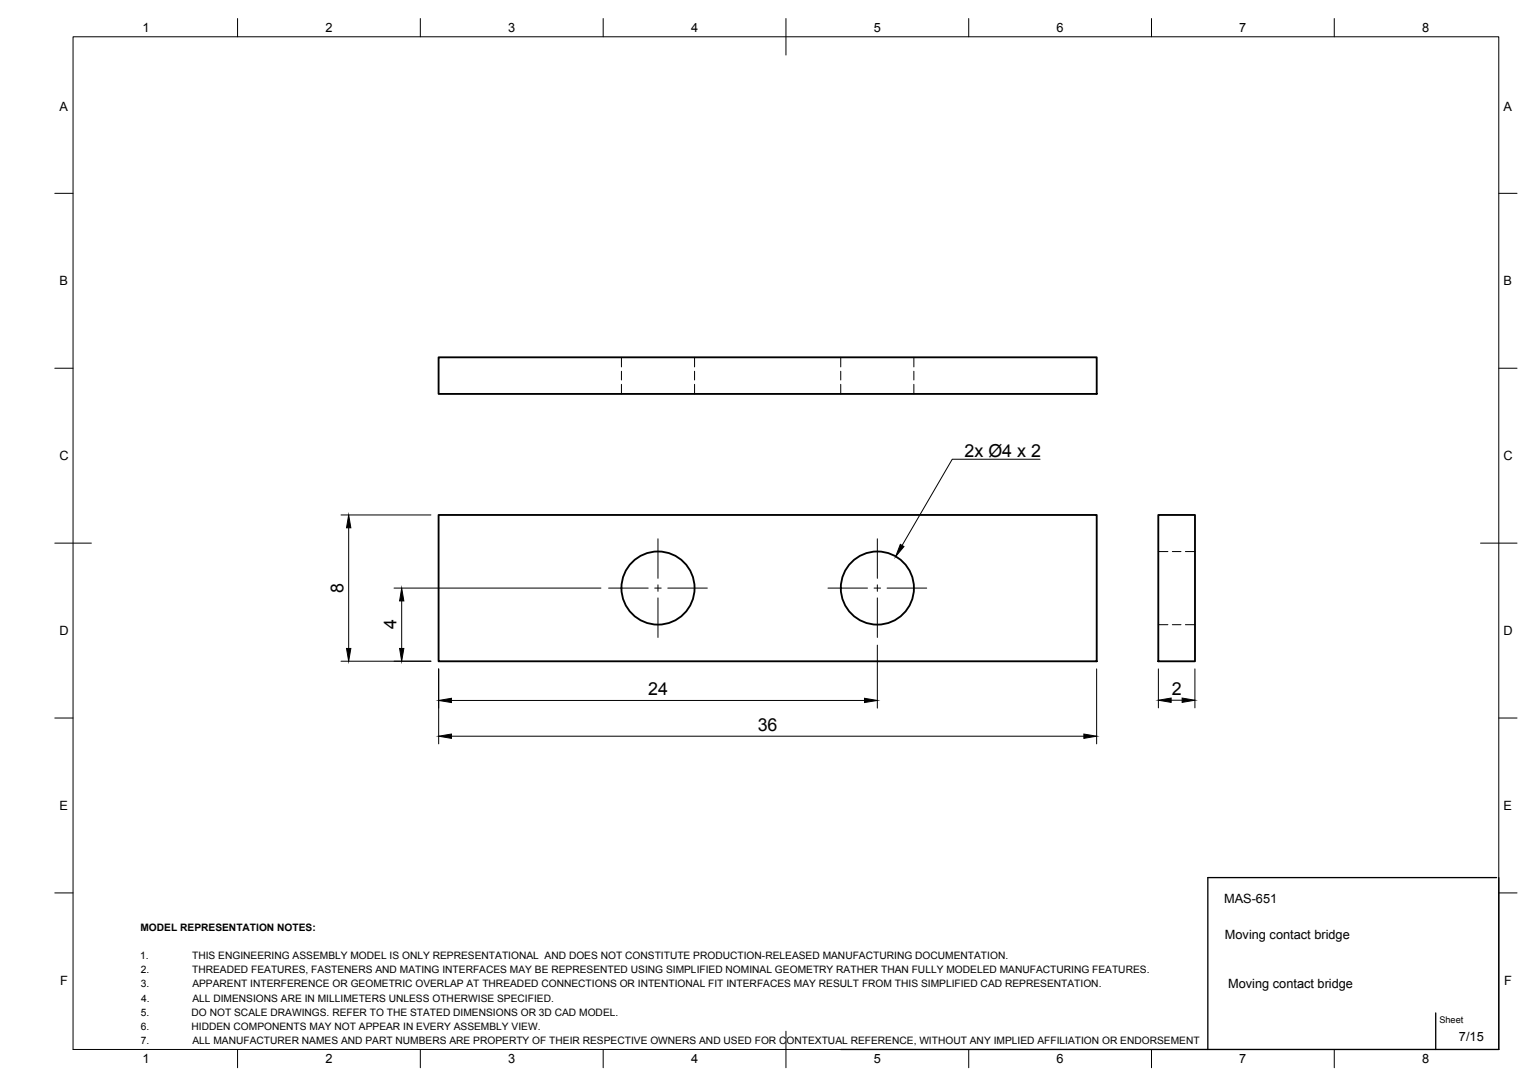
ISO-10303-21;
HEADER;
/* Generated by software containing ST-Developer
 * from STEP Tools, Inc. (www.steptools.com) 
 */

FILE_DESCRIPTION(
/* description */ ('Independent direct-acting normally-closed roller-plunger limit-switch
 CAD. Removable cover, insulated terminal supports, captured bus/conta
ct bridge, native Coil return spring, integral lower travel stop, reus
able instanced hardware and free roller. Manual geometric contact open
ing4mm; no snap-action/contact-force, electrical/current/voltage, envi
ronmental seal, safety-switch, wear, load or life certification. Exter
nal wiring and anchors omitted; fits and application engineering requi
red.'),
/* implementation_level */ '2;1');

FILE_NAME(
/* name */ 'Moving contact bridge.step',
/* time_stamp */ '2026-11-08T07:32:43-08:00',
/* author */ (''),
/* organization */ (''),
/* preprocessor_version */ 'ST-DEVELOPER v20.2',
/* originating_system */ 'Autodesk Translation Framework v15.17.0.0',
/* authorisation */ '');

FILE_SCHEMA (('AUTOMOTIVE_DESIGN { 1 0 10303 214 3 1 1 }'));
ENDSEC;

DATA;
#10=MECHANICAL_DESIGN_GEOMETRIC_PRESENTATION_REPRESENTATION('',(#180),#36482);
#146=SHAPE_REPRESENTATION_RELATIONSHIP('SRR','None',#36559,#163);
#163=ADVANCED_BREP_SHAPE_REPRESENTATION('',(#197),#36469);
#180=STYLED_ITEM('',(#36653),#197);
#197=MANIFOLD_SOLID_BREP('Body1',#9771);
#276=FACE_BOUND('',#1264,.T.);
#277=FACE_BOUND('',#1265,.T.);
#278=FACE_BOUND('',#1267,.T.);
#279=FACE_BOUND('',#1268,.T.);
#360=PLANE('',#10291);
#361=PLANE('',#10292);
#362=PLANE('',#10293);
#363=PLANE('',#10294);
#364=PLANE('',#10295);
#365=PLANE('',#10296);
#678=FACE_OUTER_BOUND('',#1257,.T.);
#679=FACE_OUTER_BOUND('',#1258,.T.);
#680=FACE_OUTER_BOUND('',#1259,.T.);
#681=FACE_OUTER_BOUND('',#1260,.T.);
#682=FACE_OUTER_BOUND('',#1261,.T.);
#683=FACE_OUTER_BOUND('',#1262,.T.);
#684=FACE_OUTER_BOUND('',#1263,.T.);
#685=FACE_OUTER_BOUND('',#1266,.T.);
#1257=EDGE_LOOP('',(#7302,#7303,#7304,#7305));
#1258=EDGE_LOOP('',(#7306,#7307,#7308,#7309));
#1259=EDGE_LOOP('',(#7310,#7311,#7312,#7313));
#1260=EDGE_LOOP('',(#7314,#7315,#7316,#7317));
#1261=EDGE_LOOP('',(#7318,#7319,#7320,#7321));
#1262=EDGE_LOOP('',(#7322,#7323,#7324,#7325));
#1263=EDGE_LOOP('',(#7326,#7327,#7328,#7329));
#1264=EDGE_LOOP('',(#7330));
#1265=EDGE_LOOP('',(#7331));
#1266=EDGE_LOOP('',(#7332,#7333,#7334,#7335));
#1267=EDGE_LOOP('',(#7336));
#1268=EDGE_LOOP('',(#7337));
#1662=CIRCLE('',#10286,0.2);
#1663=CIRCLE('',#10287,0.2);
#1664=CIRCLE('',#10289,0.2);
#1665=CIRCLE('',#10290,0.2);
#2707=LINE('',#23141,#3281);
#2708=LINE('',#23147,#3282);
#2709=LINE('',#23152,#3283);
#2710=LINE('',#23154,#3284);
#2711=LINE('',#23156,#3285);
#2712=LINE('',#23157,#3286);
#2713=LINE('',#23160,#3287);
#2714=LINE('',#23162,#3288);
#2715=LINE('',#23163,#3289);
#2716=LINE('',#23166,#3290);
#2717=LINE('',#23168,#3291);
#2718=LINE('',#23169,#3292);
#2719=LINE('',#23171,#3293);
#2720=LINE('',#23172,#3294);
#3281=VECTOR('',#11582,0.2);
#3282=VECTOR('',#11589,0.2);
#3283=VECTOR('',#11594,1.);
#3284=VECTOR('',#11595,1.);
#3285=VECTOR('',#11596,1.);
#3286=VECTOR('',#11597,1.);
#3287=VECTOR('',#11600,1.);
#3288=VECTOR('',#11601,1.);
#3289=VECTOR('',#11602,1.);
#3290=VECTOR('',#11605,1.);
#3291=VECTOR('',#11606,1.);
#3292=VECTOR('',#11607,1.);
#3293=VECTOR('',#11610,1.);
#3294=VECTOR('',#11611,1.);
#4031=VERTEX_POINT('',#23138);
#4032=VERTEX_POINT('',#23140);
#4033=VERTEX_POINT('',#23144);
#4034=VERTEX_POINT('',#23146);
#4035=VERTEX_POINT('',#23150);
#4036=VERTEX_POINT('',#23151);
#4037=VERTEX_POINT('',#23153);
#4038=VERTEX_POINT('',#23155);
#4039=VERTEX_POINT('',#23159);
#4040=VERTEX_POINT('',#23161);
#4041=VERTEX_POINT('',#23165);
#4042=VERTEX_POINT('',#23167);
#5207=EDGE_CURVE('',#4031,#4031,#1662,.T.);
#5208=EDGE_CURVE('',#4031,#4032,#2707,.T.);
#5209=EDGE_CURVE('',#4032,#4032,#1663,.T.);
#5210=EDGE_CURVE('',#4033,#4033,#1664,.T.);
#5211=EDGE_CURVE('',#4033,#4034,#2708,.T.);
#5212=EDGE_CURVE('',#4034,#4034,#1665,.T.);
#5213=EDGE_CURVE('',#4035,#4036,#2709,.T.);
#5214=EDGE_CURVE('',#4036,#4037,#2710,.T.);
#5215=EDGE_CURVE('',#4038,#4037,#2711,.T.);
#5216=EDGE_CURVE('',#4035,#4038,#2712,.T.);
#5217=EDGE_CURVE('',#4039,#4035,#2713,.T.);
#5218=EDGE_CURVE('',#4040,#4038,#2714,.T.);
#5219=EDGE_CURVE('',#4039,#4040,#2715,.T.);
#5220=EDGE_CURVE('',#4041,#4039,#2716,.T.);
#5221=EDGE_CURVE('',#4042,#4040,#2717,.T.);
#5222=EDGE_CURVE('',#4041,#4042,#2718,.T.);
#5223=EDGE_CURVE('',#4036,#4041,#2719,.T.);
#5224=EDGE_CURVE('',#4037,#4042,#2720,.T.);
#7302=ORIENTED_EDGE('',*,*,#5207,.F.);
#7303=ORIENTED_EDGE('',*,*,#5208,.T.);
#7304=ORIENTED_EDGE('',*,*,#5209,.F.);
#7305=ORIENTED_EDGE('',*,*,#5208,.F.);
#7306=ORIENTED_EDGE('',*,*,#5210,.F.);
#7307=ORIENTED_EDGE('',*,*,#5211,.T.);
#7308=ORIENTED_EDGE('',*,*,#5212,.F.);
#7309=ORIENTED_EDGE('',*,*,#5211,.F.);
#7310=ORIENTED_EDGE('',*,*,#5213,.T.);
#7311=ORIENTED_EDGE('',*,*,#5214,.T.);
#7312=ORIENTED_EDGE('',*,*,#5215,.F.);
#7313=ORIENTED_EDGE('',*,*,#5216,.F.);
#7314=ORIENTED_EDGE('',*,*,#5217,.T.);
#7315=ORIENTED_EDGE('',*,*,#5216,.T.);
#7316=ORIENTED_EDGE('',*,*,#5218,.F.);
#7317=ORIENTED_EDGE('',*,*,#5219,.F.);
#7318=ORIENTED_EDGE('',*,*,#5220,.T.);
#7319=ORIENTED_EDGE('',*,*,#5219,.T.);
#7320=ORIENTED_EDGE('',*,*,#5221,.F.);
#7321=ORIENTED_EDGE('',*,*,#5222,.F.);
#7322=ORIENTED_EDGE('',*,*,#5223,.T.);
#7323=ORIENTED_EDGE('',*,*,#5222,.T.);
#7324=ORIENTED_EDGE('',*,*,#5224,.F.);
#7325=ORIENTED_EDGE('',*,*,#5214,.F.);
#7326=ORIENTED_EDGE('',*,*,#5224,.T.);
#7327=ORIENTED_EDGE('',*,*,#5221,.T.);
#7328=ORIENTED_EDGE('',*,*,#5218,.T.);
#7329=ORIENTED_EDGE('',*,*,#5215,.T.);
#7330=ORIENTED_EDGE('',*,*,#5207,.T.);
#7331=ORIENTED_EDGE('',*,*,#5210,.T.);
#7332=ORIENTED_EDGE('',*,*,#5223,.F.);
#7333=ORIENTED_EDGE('',*,*,#5213,.F.);
#7334=ORIENTED_EDGE('',*,*,#5217,.F.);
#7335=ORIENTED_EDGE('',*,*,#5220,.F.);
#7336=ORIENTED_EDGE('',*,*,#5209,.T.);
#7337=ORIENTED_EDGE('',*,*,#5212,.T.);
#9029=CYLINDRICAL_SURFACE('',#10285,0.2);
#9030=CYLINDRICAL_SURFACE('',#10288,0.2);
#9468=ADVANCED_FACE('',(#678),#9029,.F.);
#9469=ADVANCED_FACE('',(#679),#9030,.F.);
#9470=ADVANCED_FACE('',(#680),#360,.T.);
#9471=ADVANCED_FACE('',(#681),#361,.T.);
#9472=ADVANCED_FACE('',(#682),#362,.T.);
#9473=ADVANCED_FACE('',(#683),#363,.T.);
#9474=ADVANCED_FACE('',(#684,#276,#277),#364,.T.);
#9475=ADVANCED_FACE('',(#685,#278,#279),#365,.F.);
#9771=CLOSED_SHELL('',(#9468,#9469,#9470,#9471,#9472,#9473,#9474,#9475));
#10284=AXIS2_PLACEMENT_3D('',#23136,#11576,#11577);
#10285=AXIS2_PLACEMENT_3D('',#23137,#11578,#11579);
#10286=AXIS2_PLACEMENT_3D('',#23139,#11580,#11581);
#10287=AXIS2_PLACEMENT_3D('',#23142,#11583,#11584);
#10288=AXIS2_PLACEMENT_3D('',#23143,#11585,#11586);
#10289=AXIS2_PLACEMENT_3D('',#23145,#11587,#11588);
#10290=AXIS2_PLACEMENT_3D('',#23148,#11590,#11591);
#10291=AXIS2_PLACEMENT_3D('',#23149,#11592,#11593);
#10292=AXIS2_PLACEMENT_3D('',#23158,#11598,#11599);
#10293=AXIS2_PLACEMENT_3D('',#23164,#11603,#11604);
#10294=AXIS2_PLACEMENT_3D('',#23170,#11608,#11609);
#10295=AXIS2_PLACEMENT_3D('',#23173,#11612,#11613);
#10296=AXIS2_PLACEMENT_3D('',#23174,#11614,#11615);
#11576=DIRECTION('axis',(0.,0.,1.));
#11577=DIRECTION('refdir',(1.,0.,0.));
#11578=DIRECTION('center_axis',(0.,0.,-1.));
#11579=DIRECTION('ref_axis',(1.,0.,0.));
#11580=DIRECTION('center_axis',(0.,0.,-1.));
#11581=DIRECTION('ref_axis',(1.,0.,0.));
#11582=DIRECTION('',(0.,0.,-1.));
#11583=DIRECTION('center_axis',(0.,0.,1.));
#11584=DIRECTION('ref_axis',(1.,0.,0.));
#11585=DIRECTION('center_axis',(0.,0.,-1.));
#11586=DIRECTION('ref_axis',(1.,0.,0.));
#11587=DIRECTION('center_axis',(0.,0.,-1.));
#11588=DIRECTION('ref_axis',(1.,0.,0.));
#11589=DIRECTION('',(0.,0.,-1.));
#11590=DIRECTION('center_axis',(0.,0.,1.));
#11591=DIRECTION('ref_axis',(1.,0.,0.));
#11592=DIRECTION('center_axis',(0.,1.,0.));
#11593=DIRECTION('ref_axis',(-1.,0.,0.));
#11594=DIRECTION('',(-1.,0.,0.));
#11595=DIRECTION('',(0.,0.,1.));
#11596=DIRECTION('',(-1.,0.,0.));
#11597=DIRECTION('',(0.,0.,1.));
#11598=DIRECTION('center_axis',(1.,0.,0.));
#11599=DIRECTION('ref_axis',(0.,1.,0.));
#11600=DIRECTION('',(0.,1.,0.));
#11601=DIRECTION('',(0.,1.,0.));
#11602=DIRECTION('',(0.,0.,1.));
#11603=DIRECTION('center_axis',(0.,-1.,0.));
#11604=DIRECTION('ref_axis',(1.,0.,0.));
#11605=DIRECTION('',(1.,0.,0.));
#11606=DIRECTION('',(1.,0.,0.));
#11607=DIRECTION('',(0.,0.,1.));
#11608=DIRECTION('center_axis',(-1.,0.,0.));
#11609=DIRECTION('ref_axis',(0.,-1.,0.));
#11610=DIRECTION('',(0.,-1.,0.));
#11611=DIRECTION('',(0.,-1.,0.));
#11612=DIRECTION('center_axis',(0.,0.,1.));
#11613=DIRECTION('ref_axis',(1.,0.,0.));
#11614=DIRECTION('center_axis',(0.,0.,1.));
#11615=DIRECTION('ref_axis',(1.,0.,0.));
#23136=CARTESIAN_POINT('',(0.,0.,0.));
#23137=CARTESIAN_POINT('Origin',(-0.6,1.,2.5));
#23138=CARTESIAN_POINT('',(-0.8,1.,2.6));
#23139=CARTESIAN_POINT('Origin',(-0.6,1.,2.6));
#23140=CARTESIAN_POINT('',(-0.8,1.,2.4));
#23141=CARTESIAN_POINT('',(-0.8,1.,2.5));
#23142=CARTESIAN_POINT('Origin',(-0.6,1.,2.4));
#23143=CARTESIAN_POINT('Origin',(0.6,1.,2.5));
#23144=CARTESIAN_POINT('',(0.4,1.,2.6));
#23145=CARTESIAN_POINT('Origin',(0.6,1.,2.6));
#23146=CARTESIAN_POINT('',(0.4,1.,2.4));
#23147=CARTESIAN_POINT('',(0.4,1.,2.5));
#23148=CARTESIAN_POINT('Origin',(0.6,1.,2.4));
#23149=CARTESIAN_POINT('Origin',(1.8,1.4,2.4));
#23150=CARTESIAN_POINT('',(1.8,1.4,2.4));
#23151=CARTESIAN_POINT('',(-1.8,1.4,2.4));
#23152=CARTESIAN_POINT('',(1.8,1.4,2.4));
#23153=CARTESIAN_POINT('',(-1.8,1.4,2.6));
#23154=CARTESIAN_POINT('',(-1.8,1.4,2.4));
#23155=CARTESIAN_POINT('',(1.8,1.4,2.6));
#23156=CARTESIAN_POINT('',(1.8,1.4,2.6));
#23157=CARTESIAN_POINT('',(1.8,1.4,2.4));
#23158=CARTESIAN_POINT('Origin',(1.8,0.6,2.4));
#23159=CARTESIAN_POINT('',(1.8,0.6,2.4));
#23160=CARTESIAN_POINT('',(1.8,0.6,2.4));
#23161=CARTESIAN_POINT('',(1.8,0.6,2.6));
#23162=CARTESIAN_POINT('',(1.8,0.6,2.6));
#23163=CARTESIAN_POINT('',(1.8,0.6,2.4));
#23164=CARTESIAN_POINT('Origin',(-1.8,0.6,2.4));
#23165=CARTESIAN_POINT('',(-1.8,0.6,2.4));
#23166=CARTESIAN_POINT('',(-1.8,0.6,2.4));
#23167=CARTESIAN_POINT('',(-1.8,0.6,2.6));
#23168=CARTESIAN_POINT('',(-1.8,0.6,2.6));
#23169=CARTESIAN_POINT('',(-1.8,0.6,2.4));
#23170=CARTESIAN_POINT('Origin',(-1.8,1.4,2.4));
#23171=CARTESIAN_POINT('',(-1.8,1.4,2.4));
#23172=CARTESIAN_POINT('',(-1.8,1.4,2.6));
#23173=CARTESIAN_POINT('Origin',(0.,1.,2.6));
#23174=CARTESIAN_POINT('Origin',(0.,1.,2.4));
#36450=UNCERTAINTY_MEASURE_WITH_UNIT(LENGTH_MEASURE(0.001),#36483,
'DISTANCE_ACCURACY_VALUE',
'Maximum model space distance between geometric entities at asserted c
onnectivities');
#36463=UNCERTAINTY_MEASURE_WITH_UNIT(LENGTH_MEASURE(0.001),#36483,
'DISTANCE_ACCURACY_VALUE',
'Maximum model space distance between geometric entities at asserted c
onnectivities');
#36469=(
GEOMETRIC_REPRESENTATION_CONTEXT(3)
GLOBAL_UNCERTAINTY_ASSIGNED_CONTEXT((#36450))
GLOBAL_UNIT_ASSIGNED_CONTEXT((#36483,#36485,#36486))
REPRESENTATION_CONTEXT('','3D')
);
#36482=(
GEOMETRIC_REPRESENTATION_CONTEXT(3)
GLOBAL_UNCERTAINTY_ASSIGNED_CONTEXT((#36463))
GLOBAL_UNIT_ASSIGNED_CONTEXT((#36483,#36485,#36486))
REPRESENTATION_CONTEXT('','3D')
);
#36483=(
LENGTH_UNIT()
NAMED_UNIT(*)
SI_UNIT(.CENTI.,.METRE.)
);
#36485=(
NAMED_UNIT(*)
PLANE_ANGLE_UNIT()
SI_UNIT($,.RADIAN.)
);
#36486=(
NAMED_UNIT(*)
SI_UNIT($,.STERADIAN.)
SOLID_ANGLE_UNIT()
);
#36492=SHAPE_DEFINITION_REPRESENTATION(#36510,#36559);
#36510=PRODUCT_DEFINITION_SHAPE('',$,#36578);
#36559=SHAPE_REPRESENTATION('',(#10284),#36469);
#36572=PRODUCT_DEFINITION_CONTEXT('part definition',#36628,'design');
#36578=PRODUCT_DEFINITION('Moving contact bridge',
'Moving contact bridge',#36596,#36572);
#36596=PRODUCT_DEFINITION_FORMATION('',$,#36635);
#36628=APPLICATION_CONTEXT(
'Core Data for Automotive Mechanical Design Process');
#36629=PRODUCT_CONTEXT('part definition',#36628,'mechanical');
#36635=PRODUCT('Moving contact bridge','Moving contact bridge',$,(#36629));
#36653=PRESENTATION_STYLE_ASSIGNMENT((#36667));
#36667=SURFACE_STYLE_USAGE(.BOTH.,#36681);
#36681=SURFACE_SIDE_STYLE('',(#36695));
#36695=SURFACE_STYLE_FILL_AREA(#36709);
#36709=FILL_AREA_STYLE('Contact gray',(#36723));
#36723=FILL_AREA_STYLE_COLOUR('Contact gray',#36737);
#36737=COLOUR_RGB('Contact gray',0.725490196078431,0.752941176470588,0.792156862745098);
ENDSEC;
END-ISO-10303-21;
